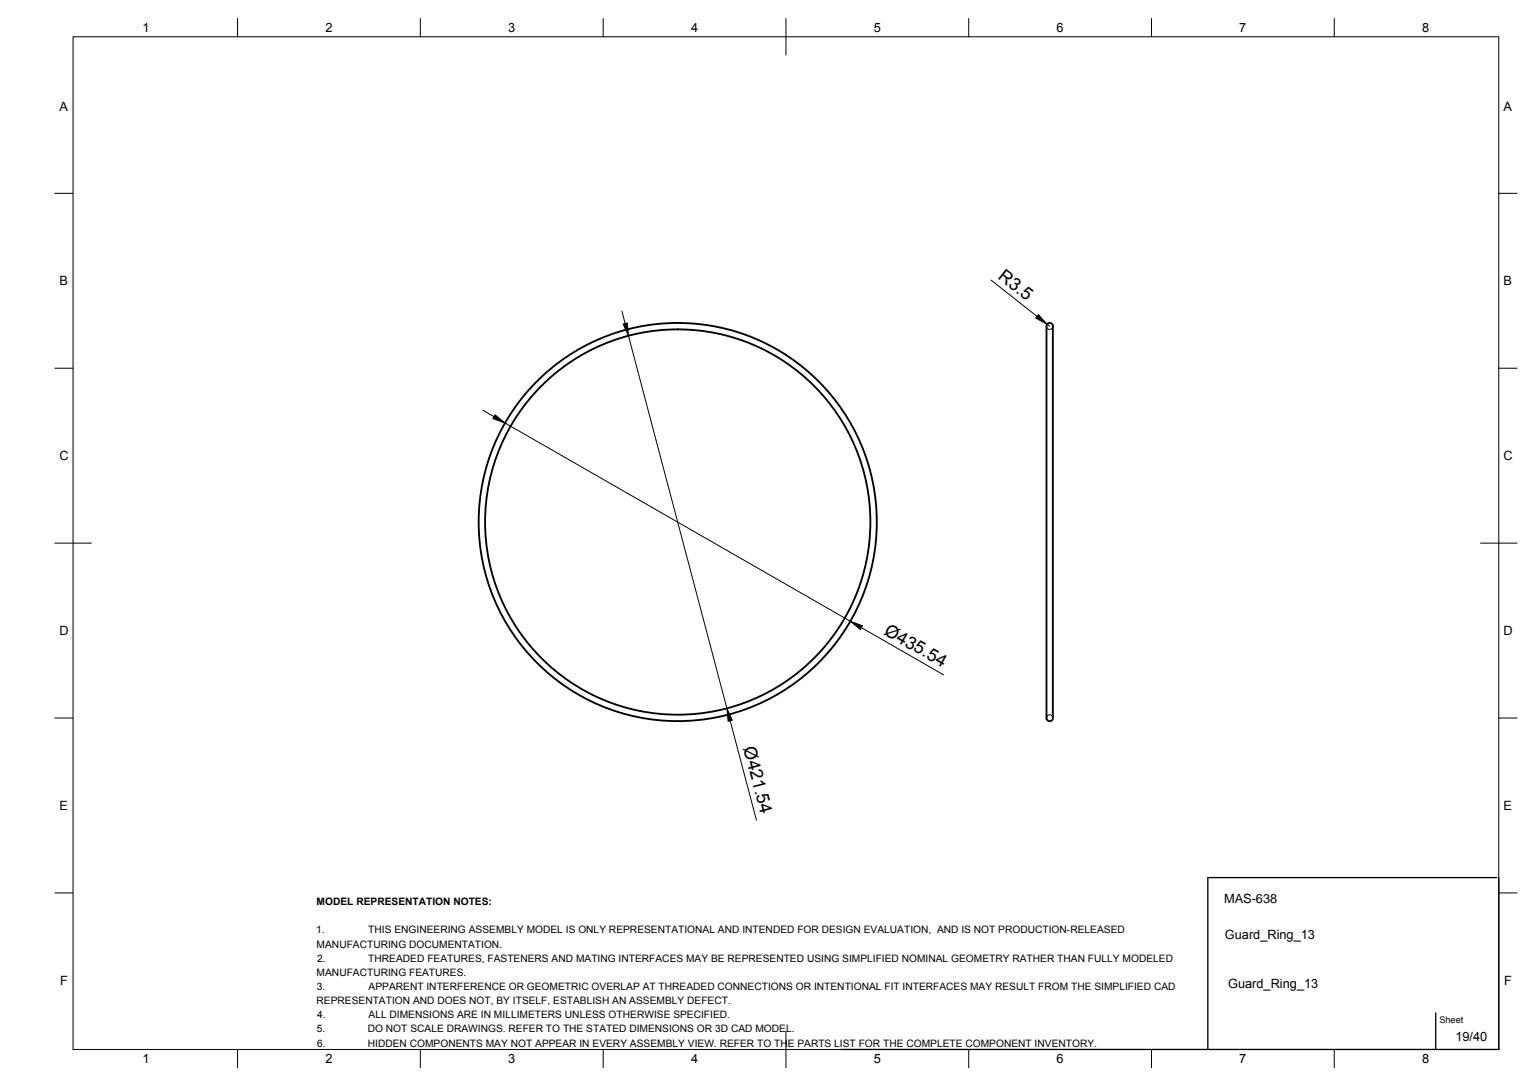
ISO-10303-21;
HEADER;
FILE_DESCRIPTION((''),'2;1');
FILE_NAME('Guard_Ring_13.step','2026-10-09T12:00:21-07:00',(''),(''),'','','');
FILE_SCHEMA (('AUTOMOTIVE_DESIGN { 1 0 10303 214 3 1 1 }'));
ENDSEC;
DATA;
#10=MECHANICAL_DESIGN_GEOMETRIC_PRESENTATION_REPRESENTATION('',(#415,#416),#10334);
#346=SHAPE_REPRESENTATION_RELATIONSHIP('SRR','None',#10462,#378) ;
#378=ADVANCED_BREP_SHAPE_REPRESENTATION('',(#450),#10314) ;
#415=STYLED_ITEM('',(#10631),#3379) ;
#416=STYLED_ITEM('',(#10632),#450) ;
#450=MANIFOLD_SOLID_BREP('Body1',#3572) ;
#871=FACE_OUTER_BOUND('',#1071,.T.) ;
#1071=EDGE_LOOP('',(#2397,#2398,#2399,#2400)) ;
#1300=CIRCLE('',#4023,0.349999999999999) ;
#1301=CIRCLE('',#4024,21.0768144613668) ;
#1525=VERTEX_POINT('',#5713) ;
#1855=EDGE_CURVE('',#1525,#1525,#1300,.T.) ;
#1856=EDGE_CURVE('',#1525,#1525,#1301,.T.) ;
#2397=ORIENTED_EDGE('',*,*,#1855,.F.) ;
#2398=ORIENTED_EDGE('',*,*,#1856,.T.) ;
#2399=ORIENTED_EDGE('',*,*,#1855,.T.) ;
#2400=ORIENTED_EDGE('',*,*,#1856,.F.) ;
#3317=TOROIDAL_SURFACE('',#4022,21.4268144613668,0.349999999999999) ;
#3379=ADVANCED_FACE('',(#871),#3317,.T.) ;
#3572=CLOSED_SHELL('',(#3379)) ;
#4021=AXIS2_PLACEMENT_3D('',#5711,#4603,#4604) ;
#4022=AXIS2_PLACEMENT_3D('',#5712,#4605,#4606) ;
#4023=AXIS2_PLACEMENT_3D('',#5714,#4607,#4608) ;
#4024=AXIS2_PLACEMENT_3D('',#5715,#4609,#4610) ;
#4603=DIRECTION('axis',(0.,0.,1.)) ;
#4604=DIRECTION('refdir',(1.,0.,0.)) ;
#4605=DIRECTION('center_axis',(-6.42891162084177E-17,-1.,-1.01883556321148E-16)) ;
#4606=DIRECTION('ref_axis',(1.,0.,0.)) ;
#4607=DIRECTION('center_axis',(0.,1.01883556321148E-16,-1.)) ;
#4608=DIRECTION('ref_axis',(-1.,0.,0.)) ;
#4609=DIRECTION('center_axis',(6.42891162084177E-17,1.,1.01883556321148E-16)) ;
#4610=DIRECTION('ref_axis',(1.,-6.42891162084177E-17,-6.55000379205715E-33)) ;
#5711=CARTESIAN_POINT('',(0.,0.,0.)) ;
#5712=CARTESIAN_POINT('Origin',(23.47768801576,67.3831179463143,68.2224337400009)) ;
#5713=CARTESIAN_POINT('',(2.4008735543932,67.3831179463143,68.2224337400009)) ;
#5714=CARTESIAN_POINT('Origin',(2.0508735543932,67.3831179463143,68.2224337400009)) ;
#5715=CARTESIAN_POINT('Origin',(23.47768801576,67.3831179463143,68.2224337400009)) ;
#10277=UNCERTAINTY_MEASURE_WITH_UNIT(LENGTH_MEASURE(0.001),#10335,
'DISTANCE_ACCURACY_VALUE',
'Maximum model space distance between geometric entities at asserted c
onnectivities') ;
#10297=UNCERTAINTY_MEASURE_WITH_UNIT(LENGTH_MEASURE(0.001),#10335,
'DISTANCE_ACCURACY_VALUE',
'Maximum model space distance between geometric entities at asserted c
onnectivities') ;
#10314=(
GEOMETRIC_REPRESENTATION_CONTEXT(3)
GLOBAL_UNCERTAINTY_ASSIGNED_CONTEXT((#10277))
GLOBAL_UNIT_ASSIGNED_CONTEXT((#10335,#10337,#10338))
REPRESENTATION_CONTEXT('','3D')
) ;
#10334=(
GEOMETRIC_REPRESENTATION_CONTEXT(3)
GLOBAL_UNCERTAINTY_ASSIGNED_CONTEXT((#10297))
GLOBAL_UNIT_ASSIGNED_CONTEXT((#10335,#10337,#10338))
REPRESENTATION_CONTEXT('','3D')
) ;
#10335=(
LENGTH_UNIT()
NAMED_UNIT(*)
SI_UNIT(.CENTI.,.METRE.)
) ;
#10337=(
NAMED_UNIT(*)
PLANE_ANGLE_UNIT()
SI_UNIT($,.RADIAN.)
) ;
#10338=(
NAMED_UNIT(*)
SI_UNIT($,.STERADIAN.)
SOLID_ANGLE_UNIT()
) ;
#10355=SHAPE_DEFINITION_REPRESENTATION(#10391,#10462) ;
#10391=PRODUCT_DEFINITION_SHAPE('',$,#10499) ;
#10462=SHAPE_REPRESENTATION('',(#4021),#10314) ;
#10482=PRODUCT_DEFINITION_CONTEXT('part definition',#10592,'design') ;
#10499=PRODUCT_DEFINITION('Guard_Ring_13','Guard_Ring_13',#10535,#10482) ;
#10535=PRODUCT_DEFINITION_FORMATION('',$,#10610) ;
#10592=APPLICATION_CONTEXT(
'Core Data for Automotive Mechanical Design Process') ;
#10593=PRODUCT_CONTEXT('part definition',#10592,'mechanical') ;
#10610=PRODUCT('Guard_Ring_13','Guard_Ring_13',$,(#10593)) ;
#10631=PRESENTATION_STYLE_ASSIGNMENT((#10635)) ;
#10632=PRESENTATION_STYLE_ASSIGNMENT((#10636)) ;
#10635=SURFACE_STYLE_USAGE(.BOTH.,#10639) ;
#10636=SURFACE_STYLE_USAGE(.BOTH.,#10640) ;
#10639=SURFACE_SIDE_STYLE('',(#10643)) ;
#10640=SURFACE_SIDE_STYLE('',(#10644)) ;
#10643=SURFACE_STYLE_FILL_AREA(#10647) ;
#10644=SURFACE_STYLE_FILL_AREA(#10648) ;
#10647=FILL_AREA_STYLE('Opaque(25,25,25)',(#10651)) ;
#10648=FILL_AREA_STYLE('Opaque(202,209,238)',(#10652)) ;
#10651=FILL_AREA_STYLE_COLOUR('Opaque(25,25,25)',#10655) ;
#10652=FILL_AREA_STYLE_COLOUR('Opaque(202,209,238)',#10656) ;
#10655=COLOUR_RGB('Opaque(25,25,25)', 0.09019608, 0.27058824, 0.51372549) ;
#10656=COLOUR_RGB('Opaque(202,209,238)', 0.40784314, 0.44705882, 0.49803922) ;
ENDSEC;
END-ISO-10303-21;
